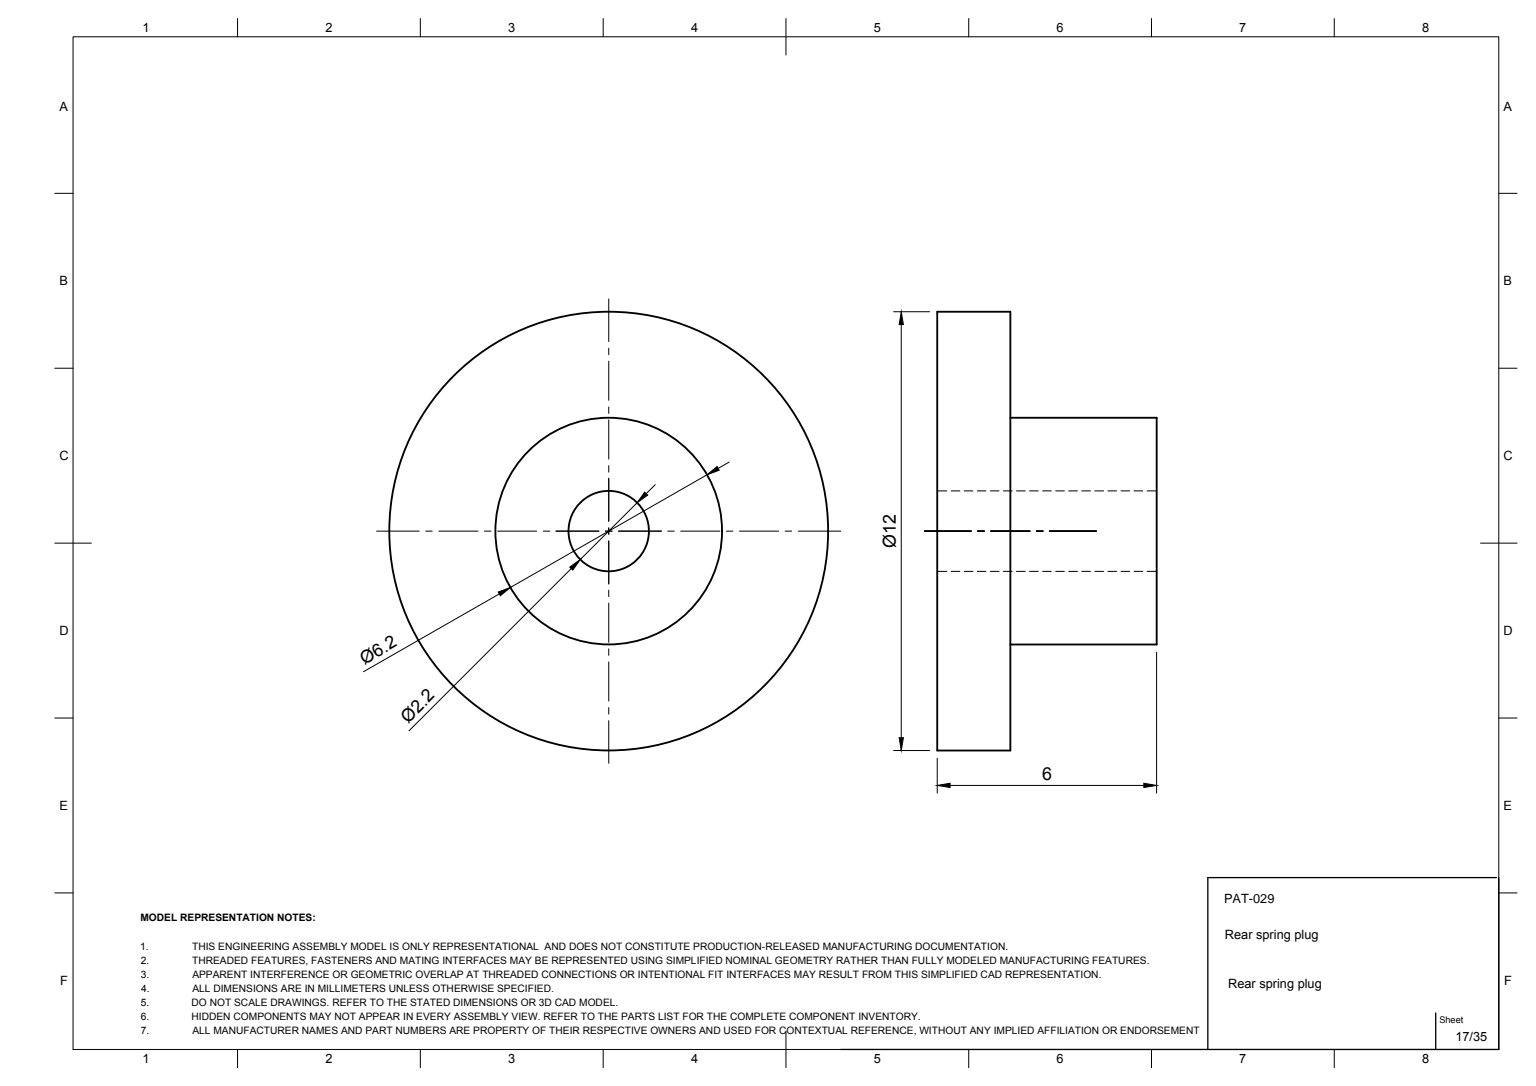
ISO-10303-21;
HEADER;
/* Generated by software containing ST-Developer
 * from STEP Tools, Inc. (www.steptools.com) 
 */

FILE_DESCRIPTION(
/* description */ ('Door-style hinge test fixture with detent'),
/* implementation_level */ '2;1');

FILE_NAME(
/* name */ 'Rear spring plug.step',
/* time_stamp */ '2026-10-28T03:24:57-07:00',
/* author */ (''),
/* organization */ (''),
/* preprocessor_version */ 'ST-DEVELOPER v20.2',
/* originating_system */ 'Autodesk Translation Framework v15.17.0.0',
/* authorisation */ '');

FILE_SCHEMA (('AUTOMOTIVE_DESIGN { 1 0 10303 214 3 1 1 }'));
ENDSEC;

DATA;
#10=MECHANICAL_DESIGN_GEOMETRIC_PRESENTATION_REPRESENTATION('',(#335),#9813);
#272=SHAPE_REPRESENTATION_RELATIONSHIP('SRR','None',#9949,#303);
#303=ADVANCED_BREP_SHAPE_REPRESENTATION('',(#375),#9792);
#335=STYLED_ITEM('',(#10183),#375);
#375=MANIFOLD_SOLID_BREP('Body1',#4766);
#460=FACE_BOUND('',#1127,.T.);
#461=FACE_BOUND('',#1130,.T.);
#462=FACE_BOUND('',#1134,.T.);
#573=PLANE('',#5369);
#574=PLANE('',#5374);
#575=PLANE('',#5380);
#780=FACE_OUTER_BOUND('',#1126,.T.);
#781=FACE_OUTER_BOUND('',#1128,.T.);
#782=FACE_OUTER_BOUND('',#1129,.T.);
#783=FACE_OUTER_BOUND('',#1131,.T.);
#784=FACE_OUTER_BOUND('',#1132,.T.);
#785=FACE_OUTER_BOUND('',#1133,.T.);
#1126=EDGE_LOOP('',(#3743));
#1127=EDGE_LOOP('',(#3744));
#1128=EDGE_LOOP('',(#3745,#3746,#3747,#3748));
#1129=EDGE_LOOP('',(#3749));
#1130=EDGE_LOOP('',(#3750));
#1131=EDGE_LOOP('',(#3751,#3752,#3753,#3754));
#1132=EDGE_LOOP('',(#3755,#3756,#3757,#3758));
#1133=EDGE_LOOP('',(#3759));
#1134=EDGE_LOOP('',(#3760));
#1503=LINE('',#7884,#1823);
#1504=LINE('',#7892,#1824);
#1505=LINE('',#7896,#1825);
#1823=VECTOR('',#6390,0.6);
#1824=VECTOR('',#6401,0.11);
#1825=VECTOR('',#6406,0.31);
#2073=CIRCLE('',#5370,0.6);
#2074=CIRCLE('',#5371,0.31);
#2075=CIRCLE('',#5373,0.6);
#2076=CIRCLE('',#5375,0.11);
#2077=CIRCLE('',#5377,0.11);
#2078=CIRCLE('',#5379,0.31);
#2401=VERTEX_POINT('',#7878);
#2402=VERTEX_POINT('',#7880);
#2403=VERTEX_POINT('',#7883);
#2404=VERTEX_POINT('',#7887);
#2405=VERTEX_POINT('',#7890);
#2406=VERTEX_POINT('',#7894);
#2888=EDGE_CURVE('',#2401,#2401,#2073,.T.);
#2889=EDGE_CURVE('',#2402,#2402,#2074,.T.);
#2890=EDGE_CURVE('',#2401,#2403,#1503,.T.);
#2891=EDGE_CURVE('',#2403,#2403,#2075,.T.);
#2892=EDGE_CURVE('',#2404,#2404,#2076,.T.);
#2893=EDGE_CURVE('',#2405,#2405,#2077,.T.);
#2894=EDGE_CURVE('',#2405,#2404,#1504,.T.);
#2895=EDGE_CURVE('',#2406,#2406,#2078,.T.);
#2896=EDGE_CURVE('',#2406,#2402,#1505,.T.);
#3743=ORIENTED_EDGE('',*,*,#2888,.T.);
#3744=ORIENTED_EDGE('',*,*,#2889,.F.);
#3745=ORIENTED_EDGE('',*,*,#2888,.F.);
#3746=ORIENTED_EDGE('',*,*,#2890,.T.);
#3747=ORIENTED_EDGE('',*,*,#2891,.T.);
#3748=ORIENTED_EDGE('',*,*,#2890,.F.);
#3749=ORIENTED_EDGE('',*,*,#2891,.F.);
#3750=ORIENTED_EDGE('',*,*,#2892,.F.);
#3751=ORIENTED_EDGE('',*,*,#2893,.F.);
#3752=ORIENTED_EDGE('',*,*,#2894,.T.);
#3753=ORIENTED_EDGE('',*,*,#2892,.T.);
#3754=ORIENTED_EDGE('',*,*,#2894,.F.);
#3755=ORIENTED_EDGE('',*,*,#2895,.F.);
#3756=ORIENTED_EDGE('',*,*,#2896,.T.);
#3757=ORIENTED_EDGE('',*,*,#2889,.T.);
#3758=ORIENTED_EDGE('',*,*,#2896,.F.);
#3759=ORIENTED_EDGE('',*,*,#2895,.T.);
#3760=ORIENTED_EDGE('',*,*,#2893,.T.);
#4424=CYLINDRICAL_SURFACE('',#5372,0.6);
#4425=CYLINDRICAL_SURFACE('',#5376,0.11);
#4426=CYLINDRICAL_SURFACE('',#5378,0.31);
#4585=ADVANCED_FACE('',(#780,#460),#573,.T.);
#4586=ADVANCED_FACE('',(#781),#4424,.T.);
#4587=ADVANCED_FACE('',(#782,#461),#574,.F.);
#4588=ADVANCED_FACE('',(#783),#4425,.F.);
#4589=ADVANCED_FACE('',(#784),#4426,.T.);
#4590=ADVANCED_FACE('',(#785,#462),#575,.T.);
#4766=CLOSED_SHELL('',(#4585,#4586,#4587,#4588,#4589,#4590));
#5368=AXIS2_PLACEMENT_3D('',#7876,#6380,#6381);
#5369=AXIS2_PLACEMENT_3D('',#7877,#6382,#6383);
#5370=AXIS2_PLACEMENT_3D('',#7879,#6384,#6385);
#5371=AXIS2_PLACEMENT_3D('',#7881,#6386,#6387);
#5372=AXIS2_PLACEMENT_3D('',#7882,#6388,#6389);
#5373=AXIS2_PLACEMENT_3D('',#7885,#6391,#6392);
#5374=AXIS2_PLACEMENT_3D('',#7886,#6393,#6394);
#5375=AXIS2_PLACEMENT_3D('',#7888,#6395,#6396);
#5376=AXIS2_PLACEMENT_3D('',#7889,#6397,#6398);
#5377=AXIS2_PLACEMENT_3D('',#7891,#6399,#6400);
#5378=AXIS2_PLACEMENT_3D('',#7893,#6402,#6403);
#5379=AXIS2_PLACEMENT_3D('',#7895,#6404,#6405);
#5380=AXIS2_PLACEMENT_3D('',#7897,#6407,#6408);
#6380=DIRECTION('axis',(0.,0.,1.));
#6381=DIRECTION('refdir',(1.,0.,0.));
#6382=DIRECTION('center_axis',(0.,1.,0.));
#6383=DIRECTION('ref_axis',(1.,0.,0.));
#6384=DIRECTION('center_axis',(0.,1.,0.));
#6385=DIRECTION('ref_axis',(1.,0.,0.));
#6386=DIRECTION('center_axis',(0.,1.,0.));
#6387=DIRECTION('ref_axis',(1.,0.,0.));
#6388=DIRECTION('center_axis',(0.,1.,0.));
#6389=DIRECTION('ref_axis',(1.,0.,0.));
#6390=DIRECTION('',(0.,-1.,0.));
#6391=DIRECTION('center_axis',(0.,1.,0.));
#6392=DIRECTION('ref_axis',(1.,0.,0.));
#6393=DIRECTION('center_axis',(0.,1.,0.));
#6394=DIRECTION('ref_axis',(1.,0.,0.));
#6395=DIRECTION('center_axis',(0.,-1.,0.));
#6396=DIRECTION('ref_axis',(1.,0.,0.));
#6397=DIRECTION('center_axis',(0.,1.,0.));
#6398=DIRECTION('ref_axis',(1.,0.,0.));
#6399=DIRECTION('center_axis',(0.,-1.,0.));
#6400=DIRECTION('ref_axis',(1.,0.,0.));
#6401=DIRECTION('',(0.,-1.,0.));
#6402=DIRECTION('center_axis',(0.,1.,0.));
#6403=DIRECTION('ref_axis',(1.,0.,0.));
#6404=DIRECTION('center_axis',(0.,1.,0.));
#6405=DIRECTION('ref_axis',(1.,0.,0.));
#6406=DIRECTION('',(0.,-1.,0.));
#6407=DIRECTION('center_axis',(0.,1.,0.));
#6408=DIRECTION('ref_axis',(1.,0.,0.));
#7876=CARTESIAN_POINT('',(0.,0.,0.));
#7877=CARTESIAN_POINT('Origin',(0.,-4.,7.2));
#7878=CARTESIAN_POINT('',(-0.6,-4.,7.2));
#7879=CARTESIAN_POINT('Origin',(0.,-4.,7.2));
#7880=CARTESIAN_POINT('',(-0.31,-4.,7.2));
#7881=CARTESIAN_POINT('Origin',(0.,-4.,7.2));
#7882=CARTESIAN_POINT('Origin',(0.,-4.2,7.2));
#7883=CARTESIAN_POINT('',(-0.6,-4.2,7.2));
#7884=CARTESIAN_POINT('',(-0.6,-4.2,7.2));
#7885=CARTESIAN_POINT('Origin',(0.,-4.2,7.2));
#7886=CARTESIAN_POINT('Origin',(0.,-4.2,7.2));
#7887=CARTESIAN_POINT('',(-0.11,-4.2,7.2));
#7888=CARTESIAN_POINT('Origin',(0.,-4.2,7.2));
#7889=CARTESIAN_POINT('Origin',(0.,-4.,7.2));
#7890=CARTESIAN_POINT('',(-0.11,-3.6,7.2));
#7891=CARTESIAN_POINT('Origin',(0.,-3.6,7.2));
#7892=CARTESIAN_POINT('',(-0.11,-4.,7.2));
#7893=CARTESIAN_POINT('Origin',(0.,-4.,7.2));
#7894=CARTESIAN_POINT('',(-0.31,-3.6,7.2));
#7895=CARTESIAN_POINT('Origin',(0.,-3.6,7.2));
#7896=CARTESIAN_POINT('',(-0.31,-4.,7.2));
#7897=CARTESIAN_POINT('Origin',(0.,-3.6,7.2));
#9756=UNCERTAINTY_MEASURE_WITH_UNIT(LENGTH_MEASURE(0.001),#9814,
'DISTANCE_ACCURACY_VALUE',
'Maximum model space distance between geometric entities at asserted c
onnectivities');
#9777=UNCERTAINTY_MEASURE_WITH_UNIT(LENGTH_MEASURE(0.001),#9814,
'DISTANCE_ACCURACY_VALUE',
'Maximum model space distance between geometric entities at asserted c
onnectivities');
#9792=(
GEOMETRIC_REPRESENTATION_CONTEXT(3)
GLOBAL_UNCERTAINTY_ASSIGNED_CONTEXT((#9756))
GLOBAL_UNIT_ASSIGNED_CONTEXT((#9814,#9816,#9817))
REPRESENTATION_CONTEXT('','3D')
);
#9813=(
GEOMETRIC_REPRESENTATION_CONTEXT(3)
GLOBAL_UNCERTAINTY_ASSIGNED_CONTEXT((#9777))
GLOBAL_UNIT_ASSIGNED_CONTEXT((#9814,#9816,#9817))
REPRESENTATION_CONTEXT('','3D')
);
#9814=(
LENGTH_UNIT()
NAMED_UNIT(*)
SI_UNIT(.CENTI.,.METRE.)
);
#9816=(
NAMED_UNIT(*)
PLANE_ANGLE_UNIT()
SI_UNIT($,.RADIAN.)
);
#9817=(
NAMED_UNIT(*)
SI_UNIT($,.STERADIAN.)
SOLID_ANGLE_UNIT()
);
#9832=SHAPE_DEFINITION_REPRESENTATION(#9867,#9949);
#9867=PRODUCT_DEFINITION_SHAPE('',$,#9985);
#9949=SHAPE_REPRESENTATION('',(#5368),#9792);
#9970=PRODUCT_DEFINITION_CONTEXT('part definition',#10077,'design');
#9985=PRODUCT_DEFINITION('Rear spring plug','Rear spring plug',#10020,#9970);
#10020=PRODUCT_DEFINITION_FORMATION('',$,#10093);
#10077=APPLICATION_CONTEXT(
'Core Data for Automotive Mechanical Design Process');
#10078=PRODUCT_CONTEXT('part definition',#10077,'mechanical');
#10093=PRODUCT('Rear spring plug','Rear spring plug','Rear spring plug',
(#10078));
#10177=COLOUR_RGB('Grey',0.48,0.52,0.57);
#10178=FILL_AREA_STYLE_COLOUR('',#10177);
#10179=FILL_AREA_STYLE('',(#10178));
#10180=SURFACE_STYLE_FILL_AREA(#10179);
#10181=SURFACE_SIDE_STYLE('',(#10180));
#10182=SURFACE_STYLE_USAGE(.BOTH.,#10181);
#10183=PRESENTATION_STYLE_ASSIGNMENT((#10182));
ENDSEC;
END-ISO-10303-21;
